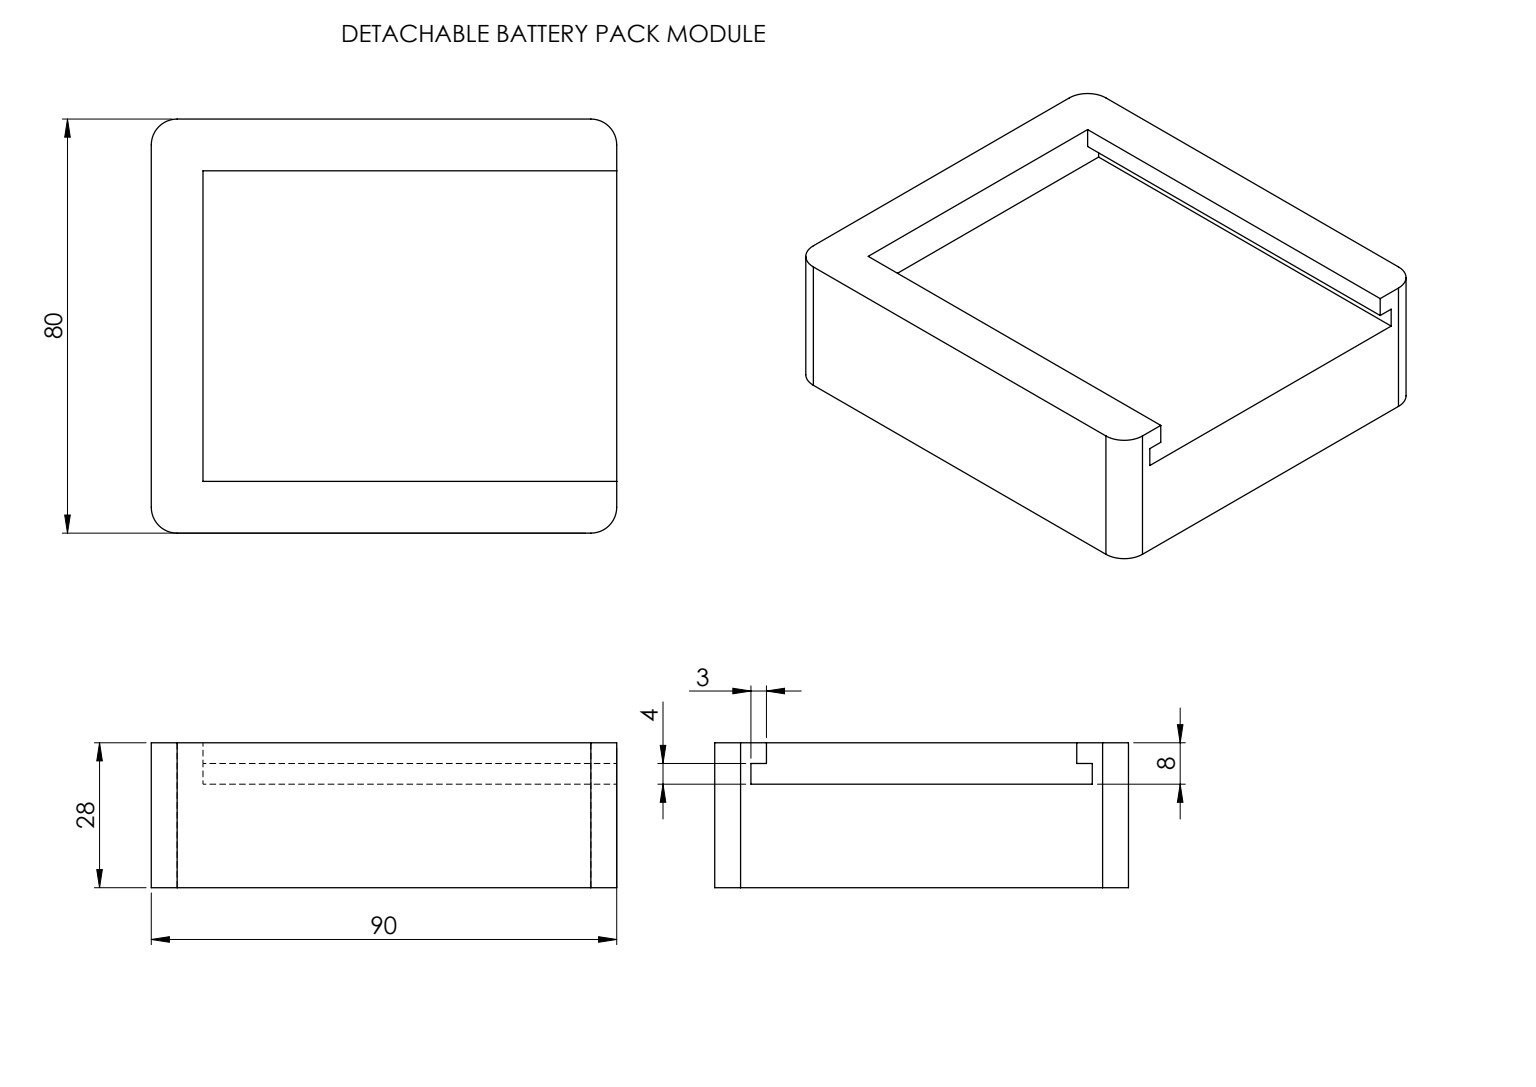
ISO-10303-21;
HEADER;
FILE_DESCRIPTION (('STEP AP214'),
    '1' );
FILE_NAME ('Detachable Battery Pack Module.step',
    '2026-10-05T20:22:16',
    ( '' ),
    ( '' ),
    'SwSTEP 2.0',
    'SolidWorks 2026',
    '' );
FILE_SCHEMA (( 'AUTOMOTIVE_DESIGN' ));
ENDSEC;

DATA;
#27=ORIENTED_EDGE ( 'NONE', *, *, #8063, .T. ) ;
#29=DIRECTION ( 'NONE',  ( 0.000000000000000000, 1.000000000000000000, 0.000000000000000000 ) ) ;
#99=ORIENTED_EDGE ( 'NONE', *, *, #10624, .F. ) ;
#105=LINE ( 'NONE', #5601, #6122 ) ;
#109=DIRECTION ( 'NONE',  ( -0.000000000000000000, -1.000000000000000000, -0.000000000000000000 ) ) ;
#122=AXIS2_PLACEMENT_3D ( 'NONE', #11876, #6482, #6572 ) ;
#131=CARTESIAN_POINT ( 'NONE',  ( 39.99999999999998579, 5.659323622547703371E-16, -33.00000000000000000 ) ) ;
#171=CARTESIAN_POINT ( 'NONE',  ( -40.00000000000000000, 8.000000000000000000, -40.00000000000000000 ) ) ;
#177=DIRECTION ( 'NONE',  ( 0.000000000000000000, -1.000000000000000000, 0.000000000000000000 ) ) ;
#268=CARTESIAN_POINT ( 'NONE',  ( 34.99999999999999289, -20.00000000000000000, 39.99999999999998579 ) ) ;
#302=EDGE_CURVE ( 'NONE', #14819, #8809, #14878, .T. ) ;
#471=LINE ( 'NONE', #14027, #16068 ) ;
#480=ORIENTED_EDGE ( 'NONE', *, *, #11200, .F. ) ;
#487=AXIS2_PLACEMENT_3D ( 'NONE', #11537, #16029, #3909 ) ;
#495=EDGE_LOOP ( 'NONE', ( #13630, #14725, #1232, #7431, #16585, #10286, #6595, #15301, #1355, #7450, #11318, #10338 ) ) ;
#526=CARTESIAN_POINT ( 'NONE',  ( 39.99999999999998579, 4.000000000000000000, -33.00000000000000000 ) ) ;
#535=EDGE_LOOP ( 'NONE', ( #5840, #7471, #16377, #3579 ) ) ;
#604=LINE ( 'NONE', #8649, #6198 ) ;
#612=EDGE_CURVE ( 'NONE', #8809, #13930, #10178, .T. ) ;
#644=ORIENTED_EDGE ( 'NONE', *, *, #1969, .F. ) ;
#648=DIRECTION ( 'NONE',  ( 8.673617379884037937E-17, -2.891205793294676354E-16, -1.000000000000000000 ) ) ;
#666=CARTESIAN_POINT ( 'NONE',  ( 39.99999999999998579, 4.000000000000000000, -33.00000000000000000 ) ) ;
#672=ORIENTED_EDGE ( 'NONE', *, *, #16461, .F. ) ;
#689=ADVANCED_FACE ( 'NONE', ( #14335 ), #14508, .T. ) ;
#753=CARTESIAN_POINT ( 'NONE',  ( -44.99999999999997868, -20.00000000000000000, 40.00000000000000711 ) ) ;
#760=AXIS2_PLACEMENT_3D ( 'NONE', #526, #3591, #2173 ) ;
#772=DIRECTION ( 'NONE',  ( -0.000000000000000000, -0.000000000000000000, 1.000000000000000000 ) ) ;
#803=( GEOMETRIC_REPRESENTATION_CONTEXT ( 3 ) GLOBAL_UNCERTAINTY_ASSIGNED_CONTEXT ( ( #9704 ) ) GLOBAL_UNIT_ASSIGNED_CONTEXT ( ( #12385, #1419, #6983 ) ) REPRESENTATION_CONTEXT ( 'NONE', 'WORKASPACE' ) );
#850=AXIS2_PLACEMENT_3D ( 'NONE', #4169, #5324, #16475 ) ;
#851=DIRECTION ( 'NONE',  ( 0.000000000000000000, -2.891205793294676354E-16, -1.000000000000000000 ) ) ;
#864=CARTESIAN_POINT ( 'NONE',  ( 39.99999999999998579, 4.000000000000000000, -33.00000000000000000 ) ) ;
#880=CARTESIAN_POINT ( 'NONE',  ( -45.00000000000000711, -20.00000000000000000, -40.00000000000000000 ) ) ;
#899=DIRECTION ( 'NONE',  ( -0.000000000000000000, -1.000000000000000000, -0.000000000000000000 ) ) ;
#925=VERTEX_POINT ( 'NONE', #11652 ) ;
#980=CARTESIAN_POINT ( 'NONE',  ( -45.00000000000001421, -20.00000000000000000, 35.00000000000000711 ) ) ;
#982=FACE_OUTER_BOUND ( 'NONE', #16917, .T. ) ;
#1076=DIRECTION ( 'NONE',  ( -1.000000000000000000, 0.000000000000000000, -8.673617379884037937E-17 ) ) ;
#1155=DIRECTION ( 'NONE',  ( 0.000000000000000000, 1.000000000000000000, 0.000000000000000000 ) ) ;
#1187=EDGE_LOOP ( 'NONE', ( #2373, #9713, #10320, #7062, #15674, #5505, #13725, #7217, #5355, #10451, #13582, #2814 ) ) ;
#1204=DIRECTION ( 'NONE',  ( -0.000000000000000000, -0.000000000000000000, 1.000000000000000000 ) ) ;
#1232=ORIENTED_EDGE ( 'NONE', *, *, #3927, .T. ) ;
#1260=AXIS2_PLACEMENT_3D ( 'NONE', #15232, #14882, #16485 ) ;
#1263=CARTESIAN_POINT ( 'NONE',  ( 34.99999999999999289, -20.00000000000000000, -35.00000000000002132 ) ) ;
#1338=CARTESIAN_POINT ( 'NONE',  ( -40.00000000000000000, 8.000000000000007105, 30.00000000000000355 ) ) ;
#1355=ORIENTED_EDGE ( 'NONE', *, *, #6344, .T. ) ;
#1372=STYLED_ITEM ( 'NONE', ( #12556 ), #2569 ) ;
#1419=( NAMED_UNIT ( * ) PLANE_ANGLE_UNIT ( ) SI_UNIT ( $, .RADIAN. ) );
#1423=DIRECTION ( 'NONE',  ( 0.000000000000000000, -0.000000000000000000, 1.000000000000000000 ) ) ;
#1424=EDGE_CURVE ( 'NONE', #8476, #8508, #15662, .T. ) ;
#1428=CYLINDRICAL_SURFACE ( 'NONE', #7596, 4.999999999999997335 ) ;
#1453=ORIENTED_EDGE ( 'NONE', *, *, #6083, .T. ) ;
#1481=VERTEX_POINT ( 'NONE', #4870 ) ;
#1498=DIRECTION ( 'NONE',  ( -1.000000000000000000, 0.000000000000000000, 0.000000000000000000 ) ) ;
#1510=EDGE_LOOP ( 'NONE', ( #13211, #4341, #7022, #15878, #8880, #5058, #3959, #10219 ) ) ;
#1555=LINE ( 'NONE', #12356, #6673 ) ;
#1556=ORIENTED_EDGE ( 'NONE', *, *, #1424, .F. ) ;
#1565=( NAMED_UNIT ( * ) SI_UNIT ( $, .STERADIAN. ) SOLID_ANGLE_UNIT ( ) );
#1585=CLOSED_SHELL ( 'NONE', ( #12508, #15158, #17233, #3535, #8065, #16357, #12591, #1655, #12803, #4422, #689, #10482, #7807, #15850, #9522, #5248, #16253, #9807 ) ) ;
#1655=ADVANCED_FACE ( 'NONE', ( #13541 ), #14946, .T. ) ;
#1662=VECTOR ( 'NONE', #12747, 1000.000000000000000 ) ;
#1663=SURFACE_STYLE_USAGE ( .BOTH. , #5645 ) ;
#1694=VECTOR ( 'NONE', #11931, 1000.000000000000000 ) ;
#1696=VERTEX_POINT ( 'NONE', #8098 ) ;
#1698=VECTOR ( 'NONE', #6202, 1000.000000000000000 ) ;
#1747=( NAMED_UNIT ( * ) PLANE_ANGLE_UNIT ( ) SI_UNIT ( $, .RADIAN. ) );
#1761=FILL_AREA_STYLE ('',( #3087 ) ) ;
#1803=VERTEX_POINT ( 'NONE', #3052 ) ;
#1804=PLANE ( 'NONE',  #16988 ) ;
#1855=EDGE_CURVE ( 'NONE', #11143, #17364, #4482, .T. ) ;
#1857=CARTESIAN_POINT ( 'NONE',  ( 39.99999999999998579, 4.000000000000007994, 33.00000000000001421 ) ) ;
#1893=DIRECTION ( 'NONE',  ( 6.938893903907229364E-16, -0.000000000000000000, -1.000000000000000000 ) ) ;
#1955=EDGE_CURVE ( 'NONE', #4989, #2572, #9262, .T. ) ;
#1969=EDGE_CURVE ( 'NONE', #1803, #9465, #6493, .T. ) ;
#2096=LINE ( 'NONE', #16729, #17441 ) ;
#2142=CARTESIAN_POINT ( 'NONE',  ( -40.00000000000000000, 4.000000000000007105, 30.00000000000000711 ) ) ;
#2173=DIRECTION ( 'NONE',  ( 1.000000000000000000, 0.000000000000000000, 8.673617379884037937E-17 ) ) ;
#2179=CARTESIAN_POINT ( 'NONE',  ( 34.99999999999999289, -20.00000000000000000, -40.00000000000001421 ) ) ;
#2196=LINE ( 'NONE', #880, #4743 ) ;
#2208=VERTEX_POINT ( 'NONE', #16049 ) ;
#2216=CARTESIAN_POINT ( 'NONE',  ( 39.99999999999997868, 8.000000000000010658, 40.00000000000000711 ) ) ;
#2243=AXIS2_PLACEMENT_3D ( 'NONE', #5868, #9754, #1076 ) ;
#2254=AXIS2_PLACEMENT_3D ( 'NONE', #12118, #6975, #8121 ) ;
#2256=VECTOR ( 'NONE', #10322, 1000.000000000000000 ) ;
#2373=ORIENTED_EDGE ( 'NONE', *, *, #6135, .T. ) ;
#2437=CARTESIAN_POINT ( 'NONE',  ( -44.99999999999998579, 8.000000000000010658, 40.00000000000000000 ) ) ;
#2452=EDGE_CURVE ( 'NONE', #9465, #8476, #4703, .T. ) ;
#2492=ORIENTED_EDGE ( 'NONE', *, *, #1855, .F. ) ;
#2498=EDGE_CURVE ( 'NONE', #10657, #14819, #17440, .T. ) ;
#2512=VECTOR ( 'NONE', #14109, 1000.000000000000000 ) ;
#2523=AXIS2_PLACEMENT_3D ( 'NONE', #6254, #15465, #11391 ) ;
#2541=DIRECTION ( 'NONE',  ( -1.000000000000000000, 0.000000000000000000, -8.673617379884037937E-17 ) ) ;
#2550=CARTESIAN_POINT ( 'NONE',  ( -40.00000000000000000, 4.000000000000000000, -33.00000000000000711 ) ) ;
#2569=ADVANCED_BREP_SHAPE_REPRESENTATION ( '', ( #5314, #3583 ), #803 ) ;
#2572=VERTEX_POINT ( 'NONE', #11945 ) ;
#2585=DIRECTION ( 'NONE',  ( 0.000000000000000000, 1.000000000000000000, 0.000000000000000000 ) ) ;
#2603=DIRECTION ( 'NONE',  ( -0.000000000000000000, -1.000000000000000000, -0.000000000000000000 ) ) ;
#2660=LINE ( 'NONE', #171, #7546 ) ;
#2662=DIRECTION ( 'NONE',  ( 7.523163845262643335E-32, 1.000000000000000000, -8.673617379884037444E-16 ) ) ;
#2671=CYLINDRICAL_SURFACE ( 'NONE', #122, 5.000000000000000888 ) ;
#2717=VERTEX_POINT ( 'NONE', #6180 ) ;
#2814=ORIENTED_EDGE ( 'NONE', *, *, #9455, .T. ) ;
#2848=EDGE_CURVE ( 'NONE', #1696, #5755, #4931, .T. ) ;
#2887=EDGE_LOOP ( 'NONE', ( #13403, #3178, #13306, #5990 ) ) ;
#2973=VERTEX_POINT ( 'NONE', #15019 ) ;
#2981=ORIENTED_EDGE ( 'NONE', *, *, #16182, .T. ) ;
#3052=CARTESIAN_POINT ( 'NONE',  ( 39.99999999999999289, 8.000000000000000000, -35.00000000000002132 ) ) ;
#3087=FILL_AREA_STYLE_COLOUR ( '', #9802 ) ;
#3137=CARTESIAN_POINT ( 'NONE',  ( 39.99999999999998579, 8.000000000000007105, 30.00000000000001066 ) ) ;
#3141=DIRECTION ( 'NONE',  ( 0.000000000000000000, 2.891205793294675861E-16, 1.000000000000000000 ) ) ;
#3178=ORIENTED_EDGE ( 'NONE', *, *, #4303, .T. ) ;
#3219=FACE_OUTER_BOUND ( 'NONE', #535, .T. ) ;
#3239=ORIENTED_EDGE ( 'NONE', *, *, #6135, .F. ) ;
#3258=DIRECTION ( 'NONE',  ( 0.000000000000000000, 1.000000000000000000, 0.000000000000000000 ) ) ;
#3274=AXIS2_PLACEMENT_3D ( 'NONE', #5480, #1498, #8297 ) ;
#3307=AXIS2_PLACEMENT_3D ( 'NONE', #15748, #14596, #11938 ) ;
#3435=AXIS2_PLACEMENT_3D ( 'NONE', #1263, #10821, #5163 ) ;
#3464=DIRECTION ( 'NONE',  ( 6.938893903907229364E-16, -3.469446951953614682E-16, -1.000000000000000000 ) ) ;
#3477=DIRECTION ( 'NONE',  ( 1.000000000000000000, -0.000000000000000000, -2.312964634635742957E-16 ) ) ;
#3504=PLANE ( 'NONE',  #14956 ) ;
#3535=ADVANCED_FACE ( 'NONE', ( #3219 ), #1804, .T. ) ;
#3546=STYLED_ITEM ( 'NONE', ( #13619 ), #5314 ) ;
#3557=EDGE_CURVE ( 'NONE', #13930, #11460, #471, .T. ) ;
#3564=EDGE_LOOP ( 'NONE', ( #3924, #13589, #644, #3850 ) ) ;
#3579=ORIENTED_EDGE ( 'NONE', *, *, #11915, .T. ) ;
#3583=AXIS2_PLACEMENT_3D ( 'NONE', #5482, #6893, #8222 ) ;
#3585=VECTOR ( 'NONE', #8683, 1000.000000000000000 ) ;
#3586=ORIENTED_EDGE ( 'NONE', *, *, #13440, .T. ) ;
#3591=DIRECTION ( 'NONE',  ( -8.673617379884037937E-17, 0.000000000000000000, 1.000000000000000000 ) ) ;
#3596=FACE_OUTER_BOUND ( 'NONE', #10262, .T. ) ;
#3619=LINE ( 'NONE', #5122, #7835 ) ;
#3640=LINE ( 'NONE', #2216, #3874 ) ;
#3684=PLANE ( 'NONE',  #760 ) ;
#3689=DIRECTION ( 'NONE',  ( -1.000000000000000000, 0.000000000000000000, -8.673617379884037937E-17 ) ) ;
#3703=FACE_OUTER_BOUND ( 'NONE', #6699, .T. ) ;
#3717=ORIENTED_EDGE ( 'NONE', *, *, #14584, .T. ) ;
#3777=CARTESIAN_POINT ( 'NONE',  ( 34.99999999999999289, 8.000000000000000000, -35.00000000000002132 ) ) ;
#3850=ORIENTED_EDGE ( 'NONE', *, *, #16742, .F. ) ;
#3851=DIRECTION ( 'NONE',  ( -2.507721281754210796E-32, -1.000000000000000000, 2.891205793294676354E-16 ) ) ;
#3874=VECTOR ( 'NONE', #3464, 1000.000000000000000 ) ;
#3897=PRODUCT_DEFINITION_FORMATION_WITH_SPECIFIED_SOURCE ( 'ANY', '', #15498, .NOT_KNOWN. ) ;
#3899=AXIS2_PLACEMENT_3D ( 'NONE', #14295, #3851, #851 ) ;
#3909=DIRECTION ( 'NONE',  ( -1.000000000000000000, 0.000000000000000000, 1.541976423090495387E-16 ) ) ;
#3913=( GEOMETRIC_REPRESENTATION_CONTEXT ( 3 ) GLOBAL_UNCERTAINTY_ASSIGNED_CONTEXT ( ( #4233 ) ) GLOBAL_UNIT_ASSIGNED_CONTEXT ( ( #5828, #12646, #4678 ) ) REPRESENTATION_CONTEXT ( 'NONE', 'WORKASPACE' ) );
#3924=ORIENTED_EDGE ( 'NONE', *, *, #7277, .F. ) ;
#3927=EDGE_CURVE ( 'NONE', #9465, #10480, #11324, .T. ) ;
#3959=ORIENTED_EDGE ( 'NONE', *, *, #7710, .F. ) ;
#3993=EDGE_CURVE ( 'NONE', #9130, #2572, #15479, .T. ) ;
#4021=ORIENTED_EDGE ( 'NONE', *, *, #11179, .T. ) ;
#4158=ORIENTED_EDGE ( 'NONE', *, *, #16909, .F. ) ;
#4169=CARTESIAN_POINT ( 'NONE',  ( 39.99999999999999289, 8.000000000000000000, -39.99999999999999289 ) ) ;
#4201=VERTEX_POINT ( 'NONE', #15021 ) ;
#4207=ORIENTED_EDGE ( 'NONE', *, *, #6451, .F. ) ;
#4233=UNCERTAINTY_MEASURE_WITH_UNIT (LENGTH_MEASURE( 1.000000000000000082E-05 ), #5828, 'distance_accuracy_value', 'NONE');
#4303=EDGE_CURVE ( 'NONE', #5755, #2973, #16626, .T. ) ;
#4321=DIRECTION ( 'NONE',  ( 0.000000000000000000, 0.000000000000000000, -1.000000000000000000 ) ) ;
#4341=ORIENTED_EDGE ( 'NONE', *, *, #11729, .F. ) ;
#4365=PLANE ( 'NONE',  #2243 ) ;
#4421=VERTEX_POINT ( 'NONE', #5908 ) ;
#4422=ADVANCED_FACE ( 'NONE', ( #10229 ), #3504, .T. ) ;
#4482=LINE ( 'NONE', #6952, #6475 ) ;
#4575=ORIENTED_EDGE ( 'NONE', *, *, #15298, .T. ) ;
#4647=CARTESIAN_POINT ( 'NONE',  ( -50.00000000000000711, -20.00000000000000000, 35.00000000000000711 ) ) ;
#4678=( NAMED_UNIT ( * ) SI_UNIT ( $, .STERADIAN. ) SOLID_ANGLE_UNIT ( ) );
#4703=LINE ( 'NONE', #10092, #1698 ) ;
#4743=VECTOR ( 'NONE', #5559, 1000.000000000000000 ) ;
#4870=CARTESIAN_POINT ( 'NONE',  ( 39.99999999999998579, -20.00000000000000000, -35.00000000000002132 ) ) ;
#4902=DIRECTION ( 'NONE',  ( 0.000000000000000000, -1.000000000000000000, 8.673617379884035472E-16 ) ) ;
#4913=FACE_OUTER_BOUND ( 'NONE', #12663, .T. ) ;
#4931=LINE ( 'NONE', #14765, #2256 ) ;
#4958=CARTESIAN_POINT ( 'NONE',  ( 34.99999999999999289, 8.000000000000000000, 34.99999999999999289 ) ) ;
#4970=ORIENTED_EDGE ( 'NONE', *, *, #11200, .T. ) ;
#4988=CARTESIAN_POINT ( 'NONE',  ( 39.99999999999998579, 8.000000000000000000, -29.99999999999999645 ) ) ;
#4989=VERTEX_POINT ( 'NONE', #10096 ) ;
#5058=ORIENTED_EDGE ( 'NONE', *, *, #12886, .F. ) ;
#5108=EDGE_CURVE ( 'NONE', #13611, #8508, #7764, .T. ) ;
#5122=CARTESIAN_POINT ( 'NONE',  ( 39.99999999999997868, 8.000000000000010658, 40.00000000000000711 ) ) ;
#5126=EDGE_CURVE ( 'NONE', #17364, #16020, #16555, .T. ) ;
#5145=DIRECTION ( 'NONE',  ( 0.000000000000000000, 0.000000000000000000, 1.000000000000000000 ) ) ;
#5152=ORIENTED_EDGE ( 'NONE', *, *, #13297, .T. ) ;
#5163=DIRECTION ( 'NONE',  ( 0.000000000000000000, 0.000000000000000000, 1.000000000000000000 ) ) ;
#5199=ORIENTED_EDGE ( 'NONE', *, *, #16103, .T. ) ;
#5248=ADVANCED_FACE ( 'NONE', ( #3703 ), #6537, .T. ) ;
#5313=DIRECTION ( 'NONE',  ( -0.000000000000000000, -1.000000000000000000, -0.000000000000000000 ) ) ;
#5314=MANIFOLD_SOLID_BREP ( 'Fillet1', #1585 ) ;
#5324=DIRECTION ( 'NONE',  ( 0.000000000000000000, 1.000000000000000000, 0.000000000000000000 ) ) ;
#5355=ORIENTED_EDGE ( 'NONE', *, *, #9268, .F. ) ;
#5434=ORIENTED_EDGE ( 'NONE', *, *, #8492, .F. ) ;
#5480=CARTESIAN_POINT ( 'NONE',  ( -50.00000000000000711, -20.00000000000000000, 40.00000000000000711 ) ) ;
#5482=CARTESIAN_POINT ( 'NONE',  ( 0.000000000000000000, 0.000000000000000000, 0.000000000000000000 ) ) ;
#5505=ORIENTED_EDGE ( 'NONE', *, *, #14789, .F. ) ;
#5559=DIRECTION ( 'NONE',  ( 0.000000000000000000, 1.000000000000000000, 0.000000000000000000 ) ) ;
#5582=ORIENTED_EDGE ( 'NONE', *, *, #10226, .T. ) ;
#5601=CARTESIAN_POINT ( 'NONE',  ( -40.00000000000000000, 4.000000000000007994, 33.00000000000000711 ) ) ;
#5621=PRODUCT_CONTEXT ( 'NONE', #8225, 'mechanical' ) ;
#5645=SURFACE_SIDE_STYLE ('',( #13694 ) ) ;
#5662=SURFACE_STYLE_FILL_AREA ( #1761 ) ;
#5682=FACE_OUTER_BOUND ( 'NONE', #10377, .T. ) ;
#5747=PLANE ( 'NONE',  #6125 ) ;
#5755=VERTEX_POINT ( 'NONE', #11364 ) ;
#5828=( LENGTH_UNIT ( ) NAMED_UNIT ( * ) SI_UNIT ( .MILLI., .METRE. ) );
#5840=ORIENTED_EDGE ( 'NONE', *, *, #16909, .T. ) ;
#5863=VECTOR ( 'NONE', #17323, 1000.000000000000000 ) ;
#5868=CARTESIAN_POINT ( 'NONE',  ( 39.99999999999998579, 4.000000000000007994, 33.00000000000001421 ) ) ;
#5871=CARTESIAN_POINT ( 'NONE',  ( 39.99999999999998579, 8.000000000000008882, 34.99999999999999289 ) ) ;
#5908=CARTESIAN_POINT ( 'NONE',  ( 39.99999999999998579, 4.000000000000000000, -30.00000000000000000 ) ) ;
#5990=ORIENTED_EDGE ( 'NONE', *, *, #12095, .T. ) ;
#6083=EDGE_CURVE ( 'NONE', #6776, #925, #105, .T. ) ;
#6122=VECTOR ( 'NONE', #29, 1000.000000000000000 ) ;
#6125=AXIS2_PLACEMENT_3D ( 'NONE', #12216, #13906, #1423 ) ;
#6135=EDGE_CURVE ( 'NONE', #2717, #1481, #9571, .T. ) ;
#6142=LINE ( 'NONE', #17472, #15017 ) ;
#6180=CARTESIAN_POINT ( 'NONE',  ( 39.99999999999998579, -20.00000000000000000, 34.99999999999999289 ) ) ;
#6198=VECTOR ( 'NONE', #772, 1000.000000000000000 ) ;
#6202=DIRECTION ( 'NONE',  ( -0.000000000000000000, -1.000000000000000000, -0.000000000000000000 ) ) ;
#6254=CARTESIAN_POINT ( 'NONE',  ( 0.000000000000000000, -20.00000000000000000, 0.000000000000000000 ) ) ;
#6280=CARTESIAN_POINT ( 'NONE',  ( 39.99999999999998579, 8.648601236627303230E-15, 33.00000000000001421 ) ) ;
#6344=EDGE_CURVE ( 'NONE', #16020, #15739, #3640, .T. ) ;
#6420=DIRECTION ( 'NONE',  ( -1.000000000000000000, 0.000000000000000000, -8.673617379884036705E-17 ) ) ;
#6425=LINE ( 'NONE', #864, #14159 ) ;
#6451=EDGE_CURVE ( 'NONE', #13930, #10657, #13763, .T. ) ;
#6465=VECTOR ( 'NONE', #7501, 1000.000000000000000 ) ;
#6475=VECTOR ( 'NONE', #9778, 1000.000000000000000 ) ;
#6482=DIRECTION ( 'NONE',  ( 0.000000000000000000, 1.000000000000000000, 0.000000000000000000 ) ) ;
#6493=CIRCLE ( 'NONE', #16405, 5.000000000000000888 ) ;
#6504=FACE_OUTER_BOUND ( 'NONE', #13919, .T. ) ;
#6513=PLANE ( 'NONE',  #16560 ) ;
#6537=CYLINDRICAL_SURFACE ( 'NONE', #7777, 4.999999999999997335 ) ;
#6572=DIRECTION ( 'NONE',  ( 0.000000000000000000, 0.000000000000000000, 1.000000000000000000 ) ) ;
#6595=ORIENTED_EDGE ( 'NONE', *, *, #13297, .F. ) ;
#6628=LINE ( 'NONE', #11930, #10435 ) ;
#6673=VECTOR ( 'NONE', #16260, 1000.000000000000000 ) ;
#6685=ORIENTED_EDGE ( 'NONE', *, *, #1424, .T. ) ;
#6699=EDGE_LOOP ( 'NONE', ( #11829, #13069, #8413, #2492 ) ) ;
#6717=ORIENTED_EDGE ( 'NONE', *, *, #16182, .F. ) ;
#6763=FACE_OUTER_BOUND ( 'NONE', #3564, .T. ) ;
#6776=VERTEX_POINT ( 'NONE', #14079 ) ;
#6893=DIRECTION ( 'NONE',  ( 0.000000000000000000, 0.000000000000000000, 1.000000000000000000 ) ) ;
#6904=VECTOR ( 'NONE', #3477, 1000.000000000000000 ) ;
#6906=DIRECTION ( 'NONE',  ( 0.000000000000000000, 1.000000000000000000, 0.000000000000000000 ) ) ;
#6928=AXIS2_PLACEMENT_3D ( 'NONE', #8934, #899, #10188 ) ;
#6947=VECTOR ( 'NONE', #648, 1000.000000000000000 ) ;
#6952=CARTESIAN_POINT ( 'NONE',  ( 34.99999999999999289, -20.00000000000000000, 39.99999999999998579 ) ) ;
#6956=PRODUCT_DEFINITION_CONTEXT ( 'detailed design', #9124, 'design' ) ;
#6975=DIRECTION ( 'NONE',  ( -8.673617379884036705E-17, -8.673617379884037444E-16, 1.000000000000000000 ) ) ;
#6983=( NAMED_UNIT ( * ) SI_UNIT ( $, .STERADIAN. ) SOLID_ANGLE_UNIT ( ) );
#7022=ORIENTED_EDGE ( 'NONE', *, *, #1955, .F. ) ;
#7040=CARTESIAN_POINT ( 'NONE',  ( 39.99999999999998579, 4.000000000000007105, 30.00000000000001421 ) ) ;
#7048=CARTESIAN_POINT ( 'NONE',  ( -40.00000000000000000, 4.000000000000007105, 30.00000000000000711 ) ) ;
#7062=ORIENTED_EDGE ( 'NONE', *, *, #12095, .F. ) ;
#7122=DIRECTION ( 'NONE',  ( 0.000000000000000000, 1.000000000000000000, -8.673617379884037444E-16 ) ) ;
#7158=SURFACE_STYLE_USAGE ( .BOTH. , #16468 ) ;
#7189=FACE_OUTER_BOUND ( 'NONE', #16403, .T. ) ;
#7217=ORIENTED_EDGE ( 'NONE', *, *, #11179, .F. ) ;
#7241=VERTEX_POINT ( 'NONE', #10994 ) ;
#7277=EDGE_CURVE ( 'NONE', #8476, #1481, #9445, .T. ) ;
#7322=ORIENTED_EDGE ( 'NONE', *, *, #2498, .T. ) ;
#7336=SHAPE_REPRESENTATION_RELATIONSHIP ( 'NONE' , 'NONE' ,  #17073, #2569 ) ;
#7348=LINE ( 'NONE', #1857, #11171 ) ;
#7431=ORIENTED_EDGE ( 'NONE', *, *, #15495, .T. ) ;
#7450=ORIENTED_EDGE ( 'NONE', *, *, #14565, .T. ) ;
#7451=LINE ( 'NONE', #12688, #6904 ) ;
#7467=CARTESIAN_POINT ( 'NONE',  ( 39.99999999999998579, 4.000000000000007105, 30.00000000000001421 ) ) ;
#7471=ORIENTED_EDGE ( 'NONE', *, *, #7710, .T. ) ;
#7501=DIRECTION ( 'NONE',  ( -1.000000000000000000, 0.000000000000000000, -8.673617379884037937E-17 ) ) ;
#7521=VECTOR ( 'NONE', #4902, 1000.000000000000000 ) ;
#7527=DIRECTION ( 'NONE',  ( 0.000000000000000000, 0.000000000000000000, 1.000000000000000000 ) ) ;
#7532=VECTOR ( 'NONE', #8248, 1000.000000000000000 ) ;
#7546=VECTOR ( 'NONE', #16213, 1000.000000000000000 ) ;
#7596=AXIS2_PLACEMENT_3D ( 'NONE', #13196, #2585, #5145 ) ;
#7600=CARTESIAN_POINT ( 'NONE',  ( 39.99999999999998579, 4.000000000000007994, 33.00000000000001421 ) ) ;
#7607=CARTESIAN_POINT ( 'NONE',  ( 39.99999999999998579, -20.00000000000000000, -40.00000000000001421 ) ) ;
#7710=EDGE_CURVE ( 'NONE', #14757, #7241, #12139, .T. ) ;
#7720=CARTESIAN_POINT ( 'NONE',  ( -50.00000000000005684, 8.000000000000000000, 35.00000000000000711 ) ) ;
#7747=LINE ( 'NONE', #12003, #13159 ) ;
#7764=CIRCLE ( 'NONE', #6928, 5.000000000000000888 ) ;
#7767=CIRCLE ( 'NONE', #10318, 5.000000000000000888 ) ;
#7775=CARTESIAN_POINT ( 'NONE',  ( -45.00000000000000711, -20.00000000000000000, 40.00000000000000711 ) ) ;
#7777=AXIS2_PLACEMENT_3D ( 'NONE', #9270, #15998, #9090 ) ;
#7807=ADVANCED_FACE ( 'NONE', ( #10881 ), #14872, .T. ) ;
#7835=VECTOR ( 'NONE', #13089, 1000.000000000000000 ) ;
#7858=CARTESIAN_POINT ( 'NONE',  ( -40.00000000000000000, 4.000000000000000000, -30.00000000000000711 ) ) ;
#7989=CYLINDRICAL_SURFACE ( 'NONE', #3435, 5.000000000000000888 ) ;
#8063=EDGE_CURVE ( 'NONE', #2973, #4989, #17250, .T. ) ;
#8065=ADVANCED_FACE ( 'NONE', ( #13270 ), #10252, .T. ) ;
#8098=CARTESIAN_POINT ( 'NONE',  ( 39.99999999999998579, 8.000000000000000000, -29.99999999999999645 ) ) ;
#8121=DIRECTION ( 'NONE',  ( 0.000000000000000000, -1.000000000000000000, -8.673617379884037444E-16 ) ) ;
#8153=ORIENTED_EDGE ( 'NONE', *, *, #2452, .T. ) ;
#8222=DIRECTION ( 'NONE',  ( 1.000000000000000000, 0.000000000000000000, 0.000000000000000000 ) ) ;
#8225=APPLICATION_CONTEXT ( 'automotive_design' ) ;
#8248=DIRECTION ( 'NONE',  ( 0.000000000000000000, 0.000000000000000000, -1.000000000000000000 ) ) ;
#8288=FILL_AREA_STYLE ('',( #13887 ) ) ;
#8297=DIRECTION ( 'NONE',  ( 0.000000000000000000, 0.000000000000000000, 1.000000000000000000 ) ) ;
#8413=ORIENTED_EDGE ( 'NONE', *, *, #5126, .F. ) ;
#8461=ORIENTED_EDGE ( 'NONE', *, *, #7277, .T. ) ;
#8472=( LENGTH_UNIT ( ) NAMED_UNIT ( * ) SI_UNIT ( .MILLI., .METRE. ) );
#8476=VERTEX_POINT ( 'NONE', #2179 ) ;
#8492=EDGE_CURVE ( 'NONE', #2208, #4989, #6425, .T. ) ;
#8508=VERTEX_POINT ( 'NONE', #11649 ) ;
#8638=MECHANICAL_DESIGN_GEOMETRIC_PRESENTATION_REPRESENTATION('',(#3546),#10614);
#8645=DIRECTION ( 'NONE',  ( 0.000000000000000000, 0.000000000000000000, -1.000000000000000000 ) ) ;
#8649=CARTESIAN_POINT ( 'NONE',  ( -50.00000000000000711, -20.00000000000000000, 40.00000000000000711 ) ) ;
#8683=DIRECTION ( 'NONE',  ( -1.000000000000000000, 0.000000000000000000, -8.673617379884037937E-17 ) ) ;
#8809=VERTEX_POINT ( 'NONE', #4647 ) ;
#8851=DIRECTION ( 'NONE',  ( 0.000000000000000000, 1.000000000000000000, 0.000000000000000000 ) ) ;
#8866=ORIENTED_EDGE ( 'NONE', *, *, #9268, .T. ) ;
#8878=LINE ( 'NONE', #17035, #7521 ) ;
#8880=ORIENTED_EDGE ( 'NONE', *, *, #4303, .F. ) ;
#8934=CARTESIAN_POINT ( 'NONE',  ( -45.00000000000000711, -20.00000000000000000, -35.00000000000000000 ) ) ;
#8952=ORIENTED_EDGE ( 'NONE', *, *, #13345, .T. ) ;
#8978=ORIENTED_EDGE ( 'NONE', *, *, #612, .T. ) ;
#8999=VECTOR ( 'NONE', #16456, 1000.000000000000000 ) ;
#9015=ORIENTED_EDGE ( 'NONE', *, *, #5108, .F. ) ;
#9022=VECTOR ( 'NONE', #14341, 1000.000000000000000 ) ;
#9070=VECTOR ( 'NONE', #3141, 1000.000000000000000 ) ;
#9090=DIRECTION ( 'NONE',  ( 0.000000000000000000, 0.000000000000000000, 1.000000000000000000 ) ) ;
#9122=DIRECTION ( 'NONE',  ( -0.000000000000000000, -1.000000000000000000, -0.000000000000000000 ) ) ;
#9124=APPLICATION_CONTEXT ( 'automotive_design' ) ;
#9130=VERTEX_POINT ( 'NONE', #131 ) ;
#9155=FACE_OUTER_BOUND ( 'NONE', #1510, .T. ) ;
#9261=ORIENTED_EDGE ( 'NONE', *, *, #13345, .F. ) ;
#9262=LINE ( 'NONE', #2550, #16964 ) ;
#9268=EDGE_CURVE ( 'NONE', #11936, #15042, #13867, .T. ) ;
#9270=CARTESIAN_POINT ( 'NONE',  ( 34.99999999999999289, -20.00000000000000000, 34.99999999999999289 ) ) ;
#9324=DIRECTION ( 'NONE',  ( -0.000000000000000000, 1.000000000000000000, 8.673617379884035472E-16 ) ) ;
#9386=FACE_OUTER_BOUND ( 'NONE', #11761, .T. ) ;
#9445=CIRCLE ( 'NONE', #17381, 5.000000000000000888 ) ;
#9455=EDGE_CURVE ( 'NONE', #16020, #2717, #6142, .T. ) ;
#9465=VERTEX_POINT ( 'NONE', #16152 ) ;
#9478=ORIENTED_EDGE ( 'NONE', *, *, #3927, .F. ) ;
#9521=EDGE_LOOP ( 'NONE', ( #2981, #10816, #5152, #7322 ) ) ;
#9522=ADVANCED_FACE ( 'NONE', ( #6763 ), #7989, .T. ) ;
#9571=LINE ( 'NONE', #14976, #7532 ) ;
#9704=UNCERTAINTY_MEASURE_WITH_UNIT (LENGTH_MEASURE( 1.000000000000000082E-05 ), #12385, 'distance_accuracy_value', 'NONE');
#9713=ORIENTED_EDGE ( 'NONE', *, *, #16742, .T. ) ;
#9754=DIRECTION ( 'NONE',  ( 8.673617379884037937E-17, 0.000000000000000000, -1.000000000000000000 ) ) ;
#9778=DIRECTION ( 'NONE',  ( 0.000000000000000000, 1.000000000000000000, 0.000000000000000000 ) ) ;
#9779=DIRECTION ( 'NONE',  ( -0.000000000000000000, 1.000000000000000000, -0.000000000000000000 ) ) ;
#9802=COLOUR_RGB ( '', 0.09019608, 0.27058824, 0.51372549) ;
#9807=ADVANCED_FACE ( 'NONE', ( #9386 ), #1428, .T. ) ;
#9861=VECTOR ( 'NONE', #9779, 1000.000000000000000 ) ;
#9931=EDGE_LOOP ( 'NONE', ( #10239, #5582, #13958, #8978 ) ) ;
#10052=CARTESIAN_POINT ( 'NONE',  ( -44.99999999999997158, 8.000000000000000000, -40.00000000000000000 ) ) ;
#10055=CARTESIAN_POINT ( 'NONE',  ( -50.00000000000000000, 8.000000000000000000, -35.00000000000000000 ) ) ;
#10092=CARTESIAN_POINT ( 'NONE',  ( 34.99999999999999289, -20.00000000000000000, -40.00000000000001421 ) ) ;
#10096=CARTESIAN_POINT ( 'NONE',  ( -40.00000000000000000, 4.000000000000000000, -33.00000000000000711 ) ) ;
#10105=ORIENTED_EDGE ( 'NONE', *, *, #5108, .T. ) ;
#10111=CARTESIAN_POINT ( 'NONE',  ( 34.99999999999999289, 8.000000000000010658, 40.00000000000000711 ) ) ;
#10178=LINE ( 'NONE', #11338, #15163 ) ;
#10187=DIRECTION ( 'NONE',  ( 0.000000000000000000, 0.000000000000000000, 1.000000000000000000 ) ) ;
#10188=DIRECTION ( 'NONE',  ( 0.000000000000000000, 0.000000000000000000, 1.000000000000000000 ) ) ;
#10219=ORIENTED_EDGE ( 'NONE', *, *, #16103, .F. ) ;
#10226=EDGE_CURVE ( 'NONE', #11460, #13611, #6628, .T. ) ;
#10229=FACE_OUTER_BOUND ( 'NONE', #1187, .T. ) ;
#10239=ORIENTED_EDGE ( 'NONE', *, *, #3557, .T. ) ;
#10252=PLANE ( 'NONE',  #2254 ) ;
#10262=EDGE_LOOP ( 'NONE', ( #1556, #8461, #3239, #4575, #6717, #16679, #99, #10105 ) ) ;
#10286=ORIENTED_EDGE ( 'NONE', *, *, #6451, .T. ) ;
#10305=DIRECTION ( 'NONE',  ( -8.673617379884036705E-17, 0.000000000000000000, 1.000000000000000000 ) ) ;
#10308=CARTESIAN_POINT ( 'NONE',  ( -50.00000000000000711, -20.00000000000000000, -35.00000000000000000 ) ) ;
#10311=LINE ( 'NONE', #17052, #14657 ) ;
#10318=AXIS2_PLACEMENT_3D ( 'NONE', #10811, #6906, #11960 ) ;
#10320=ORIENTED_EDGE ( 'NONE', *, *, #11695, .F. ) ;
#10322=DIRECTION ( 'NONE',  ( -1.000000000000000000, 0.000000000000000000, -8.673617379884037937E-17 ) ) ;
#10338=ORIENTED_EDGE ( 'NONE', *, *, #2848, .F. ) ;
#10377=EDGE_LOOP ( 'NONE', ( #11379, #27, #5434, #3717 ) ) ;
#10435=VECTOR ( 'NONE', #14590, 1000.000000000000000 ) ;
#10451=ORIENTED_EDGE ( 'NONE', *, *, #11915, .F. ) ;
#10480=VERTEX_POINT ( 'NONE', #10052 ) ;
#10482=ADVANCED_FACE ( 'NONE', ( #3596 ), #14151, .F. ) ;
#10555=LINE ( 'NONE', #4988, #12904 ) ;
#10614=( GEOMETRIC_REPRESENTATION_CONTEXT ( 3 ) GLOBAL_UNCERTAINTY_ASSIGNED_CONTEXT ( ( #15888 ) ) GLOBAL_UNIT_ASSIGNED_CONTEXT ( ( #8472, #1747, #1565 ) ) REPRESENTATION_CONTEXT ( 'NONE', 'WORKASPACE' ) );
#10624=EDGE_CURVE ( 'NONE', #13611, #8809, #604, .T. ) ;
#10657=VERTEX_POINT ( 'NONE', #2437 ) ;
#10811=CARTESIAN_POINT ( 'NONE',  ( -45.00000000000000711, 8.000000000000000000, -35.00000000000000000 ) ) ;
#10816=ORIENTED_EDGE ( 'NONE', *, *, #1855, .T. ) ;
#10821=DIRECTION ( 'NONE',  ( 0.000000000000000000, 1.000000000000000000, 0.000000000000000000 ) ) ;
#10822=DIRECTION ( 'NONE',  ( 0.000000000000000000, 0.000000000000000000, 1.000000000000000000 ) ) ;
#10881=FACE_OUTER_BOUND ( 'NONE', #495, .T. ) ;
#10974=LINE ( 'NONE', #7600, #14564 ) ;
#10994=CARTESIAN_POINT ( 'NONE',  ( -40.00000000000000711, 8.000000000000000000, 30.00000000000000711 ) ) ;
#11052=ORIENTED_EDGE ( 'NONE', *, *, #1955, .T. ) ;
#11069=PLANE ( 'NONE',  #1260 ) ;
#11143=VERTEX_POINT ( 'NONE', #268 ) ;
#11171=VECTOR ( 'NONE', #177, 1000.000000000000000 ) ;
#11179=EDGE_CURVE ( 'NONE', #15042, #4201, #7348, .T. ) ;
#11200=EDGE_CURVE ( 'NONE', #15042, #925, #10974, .T. ) ;
#11318=ORIENTED_EDGE ( 'NONE', *, *, #12886, .T. ) ;
#11324=LINE ( 'NONE', #15569, #1662 ) ;
#11338=CARTESIAN_POINT ( 'NONE',  ( -50.00000000000000711, -20.00000000000000000, 35.00000000000000711 ) ) ;
#11354=CARTESIAN_POINT ( 'NONE',  ( 39.99999999999998579, 4.000000000000007994, 33.00000000000001421 ) ) ;
#11364=CARTESIAN_POINT ( 'NONE',  ( -40.00000000000000000, 8.000000000000000000, -30.00000000000000711 ) ) ;
#11379=ORIENTED_EDGE ( 'NONE', *, *, #15094, .T. ) ;
#11391=DIRECTION ( 'NONE',  ( 0.000000000000000000, -0.000000000000000000, 1.000000000000000000 ) ) ;
#11414=LINE ( 'NONE', #6280, #3585 ) ;
#11460=VERTEX_POINT ( 'NONE', #10055 ) ;
#11537=CARTESIAN_POINT ( 'NONE',  ( 39.99999999999998579, -20.00000000000000000, -40.00000000000001421 ) ) ;
#11649=CARTESIAN_POINT ( 'NONE',  ( -44.99999999999997868, -20.00000000000000000, -40.00000000000000000 ) ) ;
#11650=CARTESIAN_POINT ( 'NONE',  ( 39.99999999999998579, 8.000000000000007105, 30.00000000000001066 ) ) ;
#11652=CARTESIAN_POINT ( 'NONE',  ( -40.00000000000000000, 4.000000000000007994, 33.00000000000001421 ) ) ;
#11695=EDGE_CURVE ( 'NONE', #1696, #1803, #7747, .T. ) ;
#11729=EDGE_CURVE ( 'NONE', #2572, #6776, #1555, .T. ) ;
#11761=EDGE_LOOP ( 'NONE', ( #13734, #12081, #4207, #15357 ) ) ;
#11766=CARTESIAN_POINT ( 'NONE',  ( -45.00000000000001421, 8.000000000000000000, 35.00000000000000711 ) ) ;
#11829=ORIENTED_EDGE ( 'NONE', *, *, #15298, .F. ) ;
#11876=CARTESIAN_POINT ( 'NONE',  ( -45.00000000000000711, -20.00000000000000000, -35.00000000000000000 ) ) ;
#11915=EDGE_CURVE ( 'NONE', #15739, #11936, #8878, .T. ) ;
#11919=DIRECTION ( 'NONE',  ( 0.000000000000000000, 0.000000000000000000, 1.000000000000000000 ) ) ;
#11930=CARTESIAN_POINT ( 'NONE',  ( -50.00000000000000711, -20.00000000000000000, -35.00000000000000000 ) ) ;
#11931=DIRECTION ( 'NONE',  ( 8.673617379884037937E-17, 0.000000000000000000, -1.000000000000000000 ) ) ;
#11936=VERTEX_POINT ( 'NONE', #7467 ) ;
#11938=DIRECTION ( 'NONE',  ( 1.000000000000000000, 0.000000000000000000, -2.312964634635742957E-16 ) ) ;
#11945=CARTESIAN_POINT ( 'NONE',  ( -39.99999999999997158, 5.659323622547703371E-16, -33.00000000000000711 ) ) ;
#11960=DIRECTION ( 'NONE',  ( 0.000000000000000000, 0.000000000000000000, 1.000000000000000000 ) ) ;
#12003=CARTESIAN_POINT ( 'NONE',  ( 39.99999999999999289, 8.000000000000000000, -39.99999999999999289 ) ) ;
#12008=LINE ( 'NONE', #13257, #5863 ) ;
#12009=DIRECTION ( 'NONE',  ( 0.000000000000000000, -1.000000000000000000, 0.000000000000000000 ) ) ;
#12061=AXIS2_PLACEMENT_3D ( 'NONE', #11766, #8851, #10187 ) ;
#12081=ORIENTED_EDGE ( 'NONE', *, *, #2498, .F. ) ;
#12095=EDGE_CURVE ( 'NONE', #4421, #1696, #10555, .T. ) ;
#12118=CARTESIAN_POINT ( 'NONE',  ( 39.99999999999998579, 8.000000000000000000, -29.99999999999999645 ) ) ;
#12139=LINE ( 'NONE', #1338, #12158 ) ;
#12158=VECTOR ( 'NONE', #2662, 1000.000000000000000 ) ;
#12216=CARTESIAN_POINT ( 'NONE',  ( 0.000000000000000000, 0.000000000000000000, 0.000000000000000000 ) ) ;
#12239=CARTESIAN_POINT ( 'NONE',  ( 34.99999999999999289, -20.00000000000000000, -35.00000000000002132 ) ) ;
#12295=AXIS2_PLACEMENT_3D ( 'NONE', #4958, #1155, #7527 ) ;
#12356=CARTESIAN_POINT ( 'NONE',  ( -40.00000000000000000, 0.000000000000000000, -40.00000000000000000 ) ) ;
#12357=EDGE_LOOP ( 'NONE', ( #13174, #15785, #672, #3586 ) ) ;
#12385=( LENGTH_UNIT ( ) NAMED_UNIT ( * ) SI_UNIT ( .MILLI., .METRE. ) );
#12508=ADVANCED_FACE ( 'NONE', ( #16388 ), #5747, .T. ) ;
#12556=PRESENTATION_STYLE_ASSIGNMENT (( #7158 ) ) ;
#12591=ADVANCED_FACE ( 'NONE', ( #4913 ), #3684, .T. ) ;
#12614=LINE ( 'NONE', #666, #9861 ) ;
#12646=( NAMED_UNIT ( * ) PLANE_ANGLE_UNIT ( ) SI_UNIT ( $, .RADIAN. ) );
#12663=EDGE_LOOP ( 'NONE', ( #14472, #11052, #13504, #17338 ) ) ;
#12688=CARTESIAN_POINT ( 'NONE',  ( 39.99999999999998579, -20.00000000000000000, 39.99999999999998579 ) ) ;
#12747=DIRECTION ( 'NONE',  ( -1.000000000000000000, 0.000000000000000000, -8.673617379884037937E-17 ) ) ;
#12803=ADVANCED_FACE ( 'NONE', ( #12867 ), #14279, .T. ) ;
#12867=FACE_OUTER_BOUND ( 'NONE', #16398, .T. ) ;
#12886=EDGE_CURVE ( 'NONE', #7241, #5755, #2660, .T. ) ;
#12904=VECTOR ( 'NONE', #9324, 1000.000000000000000 ) ;
#12921=ORIENTED_EDGE ( 'NONE', *, *, #15495, .F. ) ;
#12980=CARTESIAN_POINT ( 'NONE',  ( 39.99999999999998579, -20.00000000000000000, 39.99999999999998579 ) ) ;
#13010=DIRECTION ( 'NONE',  ( -1.000000000000000000, 0.000000000000000000, -8.673617379884037937E-17 ) ) ;
#13069=ORIENTED_EDGE ( 'NONE', *, *, #9455, .F. ) ;
#13089=DIRECTION ( 'NONE',  ( -1.000000000000000000, 0.000000000000000000, -8.673617379884037937E-17 ) ) ;
#13147=CARTESIAN_POINT ( 'NONE',  ( -40.00000000000000711, 0.000000000000000000, -3.469446951953615767E-15 ) ) ;
#13159=VECTOR ( 'NONE', #17407, 1000.000000000000000 ) ;
#13174=ORIENTED_EDGE ( 'NONE', *, *, #3993, .T. ) ;
#13196=CARTESIAN_POINT ( 'NONE',  ( -45.00000000000001421, -20.00000000000000000, 35.00000000000000711 ) ) ;
#13211=ORIENTED_EDGE ( 'NONE', *, *, #6083, .F. ) ;
#13257=CARTESIAN_POINT ( 'NONE',  ( 39.99999999999998579, 4.000000000000007105, 30.00000000000001421 ) ) ;
#13270=FACE_OUTER_BOUND ( 'NONE', #2887, .T. ) ;
#13297=EDGE_CURVE ( 'NONE', #17364, #10657, #3619, .T. ) ;
#13306=ORIENTED_EDGE ( 'NONE', *, *, #15094, .F. ) ;
#13345=EDGE_CURVE ( 'NONE', #8508, #10480, #2196, .T. ) ;
#13403=ORIENTED_EDGE ( 'NONE', *, *, #2848, .T. ) ;
#13440=EDGE_CURVE ( 'NONE', #4201, #9130, #16458, .T. ) ;
#13504=ORIENTED_EDGE ( 'NONE', *, *, #3993, .F. ) ;
#13541=FACE_OUTER_BOUND ( 'NONE', #9931, .T. ) ;
#13582=ORIENTED_EDGE ( 'NONE', *, *, #6344, .F. ) ;
#13589=ORIENTED_EDGE ( 'NONE', *, *, #2452, .F. ) ;
#13595=SHAPE_DEFINITION_REPRESENTATION ( #16346, #17073 ) ;
#13611=VERTEX_POINT ( 'NONE', #10308 ) ;
#13619=PRESENTATION_STYLE_ASSIGNMENT (( #1663 ) ) ;
#13630=ORIENTED_EDGE ( 'NONE', *, *, #11695, .T. ) ;
#13694=SURFACE_STYLE_FILL_AREA ( #8288 ) ;
#13725=ORIENTED_EDGE ( 'NONE', *, *, #13440, .F. ) ;
#13734=ORIENTED_EDGE ( 'NONE', *, *, #302, .F. ) ;
#13753=LINE ( 'NONE', #16765, #2512 ) ;
#13763=CIRCLE ( 'NONE', #12061, 4.999999999999997335 ) ;
#13867=LINE ( 'NONE', #7040, #9070 ) ;
#13887=FILL_AREA_STYLE_COLOUR ( '', #17110 ) ;
#13906=DIRECTION ( 'NONE',  ( 0.000000000000000000, 1.000000000000000000, 0.000000000000000000 ) ) ;
#13919=EDGE_LOOP ( 'NONE', ( #4970, #5199, #4158, #8866 ) ) ;
#13930=VERTEX_POINT ( 'NONE', #7720 ) ;
#13958=ORIENTED_EDGE ( 'NONE', *, *, #10624, .T. ) ;
#13996=DIRECTION ( 'NONE',  ( 0.000000000000000000, 1.000000000000000000, 0.000000000000000000 ) ) ;
#14027=CARTESIAN_POINT ( 'NONE',  ( -50.00000000000000000, 8.000000000000000000, -40.00000000000000000 ) ) ;
#14079=CARTESIAN_POINT ( 'NONE',  ( -40.00000000000000711, 0.000000000000000000, 33.00000000000000711 ) ) ;
#14109=DIRECTION ( 'NONE',  ( -1.000000000000000000, 0.000000000000000000, -8.673617379884037937E-17 ) ) ;
#14151=PLANE ( 'NONE',  #2523 ) ;
#14159=VECTOR ( 'NONE', #3689, 1000.000000000000000 ) ;
#14194=CARTESIAN_POINT ( 'NONE',  ( 34.99999999999999289, -20.00000000000000000, 34.99999999999999289 ) ) ;
#14279=PLANE ( 'NONE',  #487 ) ;
#14295=CARTESIAN_POINT ( 'NONE',  ( 39.99999999999998579, 4.000000000000007105, 30.00000000000001421 ) ) ;
#14320=AXIS2_PLACEMENT_3D ( 'NONE', #980, #16140, #14718 ) ;
#14335=FACE_OUTER_BOUND ( 'NONE', #9521, .T. ) ;
#14341=DIRECTION ( 'NONE',  ( -1.000000000000000000, 0.000000000000000000, 1.541976423090495387E-16 ) ) ;
#14406=CIRCLE ( 'NONE', #16111, 4.999999999999997335 ) ;
#14472=ORIENTED_EDGE ( 'NONE', *, *, #8492, .T. ) ;
#14508=PLANE ( 'NONE',  #3307 ) ;
#14525=DIRECTION ( 'NONE',  ( 0.000000000000000000, 0.000000000000000000, 1.000000000000000000 ) ) ;
#14564=VECTOR ( 'NONE', #13010, 1000.000000000000000 ) ;
#14565=EDGE_CURVE ( 'NONE', #15739, #7241, #17134, .T. ) ;
#14584=EDGE_CURVE ( 'NONE', #2208, #4421, #10311, .T. ) ;
#14590=DIRECTION ( 'NONE',  ( -0.000000000000000000, -1.000000000000000000, -0.000000000000000000 ) ) ;
#14596=DIRECTION ( 'NONE',  ( 2.312964634635742957E-16, -0.000000000000000000, 1.000000000000000000 ) ) ;
#14657=VECTOR ( 'NONE', #1204, 1000.000000000000000 ) ;
#14718=DIRECTION ( 'NONE',  ( 0.000000000000000000, 0.000000000000000000, 1.000000000000000000 ) ) ;
#14725=ORIENTED_EDGE ( 'NONE', *, *, #1969, .T. ) ;
#14757=VERTEX_POINT ( 'NONE', #7048 ) ;
#14765=CARTESIAN_POINT ( 'NONE',  ( 39.99999999999998579, 8.000000000000000000, -29.99999999999999645 ) ) ;
#14769=ORIENTED_EDGE ( 'NONE', *, *, #16461, .T. ) ;
#14789=EDGE_CURVE ( 'NONE', #9130, #2208, #12614, .T. ) ;
#14819=VERTEX_POINT ( 'NONE', #753 ) ;
#14827=ORIENTED_EDGE ( 'NONE', *, *, #10226, .F. ) ;
#14843=CARTESIAN_POINT ( 'NONE',  ( -40.00000000000000000, 8.000000000000000000, -30.00000000000000355 ) ) ;
#14846=CARTESIAN_POINT ( 'NONE',  ( 39.99999999999998579, 0.000000000000000000, 39.99999999999998579 ) ) ;
#14872=PLANE ( 'NONE',  #850 ) ;
#14878=CIRCLE ( 'NONE', #14320, 4.999999999999997335 ) ;
#14882=DIRECTION ( 'NONE',  ( 0.000000000000000000, -1.000000000000000000, 0.000000000000000000 ) ) ;
#14946=PLANE ( 'NONE',  #3274 ) ;
#14956=AXIS2_PLACEMENT_3D ( 'NONE', #12980, #15548, #8645 ) ;
#14976=CARTESIAN_POINT ( 'NONE',  ( 39.99999999999998579, -20.00000000000000000, 39.99999999999998579 ) ) ;
#15017=VECTOR ( 'NONE', #2603, 1000.000000000000000 ) ;
#15019=CARTESIAN_POINT ( 'NONE',  ( -40.00000000000000000, 4.000000000000000000, -30.00000000000000000 ) ) ;
#15021=CARTESIAN_POINT ( 'NONE',  ( 39.99999999999998579, 0.000000000000000000, 33.00000000000001421 ) ) ;
#15042=VERTEX_POINT ( 'NONE', #11354 ) ;
#15094=EDGE_CURVE ( 'NONE', #4421, #2973, #13753, .T. ) ;
#15158=ADVANCED_FACE ( 'NONE', ( #7189 ), #4365, .T. ) ;
#15163=VECTOR ( 'NONE', #13996, 1000.000000000000000 ) ;
#15232=CARTESIAN_POINT ( 'NONE',  ( 39.99999999999998579, 4.000000000000000000, -30.00000000000000000 ) ) ;
#15298=EDGE_CURVE ( 'NONE', #2717, #11143, #14406, .T. ) ;
#15301=ORIENTED_EDGE ( 'NONE', *, *, #5126, .T. ) ;
#15344=DIRECTION ( 'NONE',  ( 8.673617379884036705E-17, -8.673617379884037444E-16, -1.000000000000000000 ) ) ;
#15357=ORIENTED_EDGE ( 'NONE', *, *, #612, .F. ) ;
#15384=CARTESIAN_POINT ( 'NONE',  ( 39.99999999999998579, 5.659323622547703371E-16, -33.00000000000000000 ) ) ;
#15465=DIRECTION ( 'NONE',  ( 0.000000000000000000, 1.000000000000000000, 0.000000000000000000 ) ) ;
#15479=LINE ( 'NONE', #15384, #6465 ) ;
#15495=EDGE_CURVE ( 'NONE', #10480, #11460, #7767, .T. ) ;
#15498=PRODUCT ( 'Detachable Battery Pack Module', 'Detachable Battery Pack Module', '', ( #5621 ) ) ;
#15548=DIRECTION ( 'NONE',  ( 1.000000000000000000, -0.000000000000000000, 0.000000000000000000 ) ) ;
#15569=CARTESIAN_POINT ( 'NONE',  ( 39.99999999999999289, 8.000000000000000000, -39.99999999999999289 ) ) ;
#15662=LINE ( 'NONE', #7607, #9022 ) ;
#15674=ORIENTED_EDGE ( 'NONE', *, *, #14584, .F. ) ;
#15739=VERTEX_POINT ( 'NONE', #16796 ) ;
#15748=CARTESIAN_POINT ( 'NONE',  ( 39.99999999999998579, -20.00000000000000000, 39.99999999999998579 ) ) ;
#15785=ORIENTED_EDGE ( 'NONE', *, *, #11729, .T. ) ;
#15850=ADVANCED_FACE ( 'NONE', ( #9155 ), #6513, .F. ) ;
#15878=ORIENTED_EDGE ( 'NONE', *, *, #8063, .F. ) ;
#15888=UNCERTAINTY_MEASURE_WITH_UNIT (LENGTH_MEASURE( 1.000000000000000082E-05 ), #8472, 'distance_accuracy_value', 'NONE');
#15971=PLANE ( 'NONE',  #3899 ) ;
#15998=DIRECTION ( 'NONE',  ( 0.000000000000000000, 1.000000000000000000, 0.000000000000000000 ) ) ;
#16020=VERTEX_POINT ( 'NONE', #5871 ) ;
#16029=DIRECTION ( 'NONE',  ( -1.541976423090495387E-16, 0.000000000000000000, -1.000000000000000000 ) ) ;
#16049=CARTESIAN_POINT ( 'NONE',  ( 39.99999999999998579, 4.000000000000000000, -33.00000000000000000 ) ) ;
#16068=VECTOR ( 'NONE', #1893, 1000.000000000000000 ) ;
#16103=EDGE_CURVE ( 'NONE', #925, #14757, #16590, .T. ) ;
#16111=AXIS2_PLACEMENT_3D ( 'NONE', #14194, #9122, #14525 ) ;
#16140=DIRECTION ( 'NONE',  ( -0.000000000000000000, -1.000000000000000000, -0.000000000000000000 ) ) ;
#16152=CARTESIAN_POINT ( 'NONE',  ( 34.99999999999999289, 8.000000000000000000, -39.99999999999999289 ) ) ;
#16182=EDGE_CURVE ( 'NONE', #14819, #11143, #7451, .T. ) ;
#16213=DIRECTION ( 'NONE',  ( 8.673617379884036705E-17, -0.000000000000000000, -1.000000000000000000 ) ) ;
#16253=ADVANCED_FACE ( 'NONE', ( #982 ), #2671, .T. ) ;
#16260=DIRECTION ( 'NONE',  ( -8.673617379884036705E-17, 0.000000000000000000, 1.000000000000000000 ) ) ;
#16346=PRODUCT_DEFINITION_SHAPE ( 'NONE', 'NONE',  #17347 ) ;
#16357=ADVANCED_FACE ( 'NONE', ( #5682 ), #11069, .T. ) ;
#16374=VECTOR ( 'NONE', #2541, 1000.000000000000000 ) ;
#16377=ORIENTED_EDGE ( 'NONE', *, *, #14565, .F. ) ;
#16388=FACE_OUTER_BOUND ( 'NONE', #12357, .T. ) ;
#16398=EDGE_LOOP ( 'NONE', ( #9478, #8153, #6685, #8952 ) ) ;
#16403=EDGE_LOOP ( 'NONE', ( #14769, #1453, #480, #4021 ) ) ;
#16405=AXIS2_PLACEMENT_3D ( 'NONE', #3777, #17237, #11919 ) ;
#16417=VECTOR ( 'NONE', #5313, 1000.000000000000000 ) ;
#16456=DIRECTION ( 'NONE',  ( 7.523163845262643335E-32, -1.000000000000000000, -8.673617379884037444E-16 ) ) ;
#16458=LINE ( 'NONE', #14846, #17468 ) ;
#16461=EDGE_CURVE ( 'NONE', #4201, #6776, #11414, .T. ) ;
#16468=SURFACE_SIDE_STYLE ('',( #5662 ) ) ;
#16475=DIRECTION ( 'NONE',  ( 0.000000000000000000, -0.000000000000000000, 1.000000000000000000 ) ) ;
#16485=DIRECTION ( 'NONE',  ( 0.000000000000000000, 0.000000000000000000, -1.000000000000000000 ) ) ;
#16555=CIRCLE ( 'NONE', #12295, 4.999999999999997335 ) ;
#16560=AXIS2_PLACEMENT_3D ( 'NONE', #13147, #6420, #10305 ) ;
#16585=ORIENTED_EDGE ( 'NONE', *, *, #3557, .F. ) ;
#16590=LINE ( 'NONE', #2142, #6947 ) ;
#16598=MECHANICAL_DESIGN_GEOMETRIC_PRESENTATION_REPRESENTATION('',(#1372),#3913);
#16626=LINE ( 'NONE', #14843, #8999 ) ;
#16679=ORIENTED_EDGE ( 'NONE', *, *, #302, .T. ) ;
#16729=CARTESIAN_POINT ( 'NONE',  ( 39.99999999999998579, -20.00000000000000000, -35.00000000000002132 ) ) ;
#16742=EDGE_CURVE ( 'NONE', #1481, #1803, #2096, .T. ) ;
#16765=CARTESIAN_POINT ( 'NONE',  ( 39.99999999999998579, 4.000000000000000000, -30.00000000000000000 ) ) ;
#16796=CARTESIAN_POINT ( 'NONE',  ( 39.99999999999998579, 8.000000000000007105, 30.00000000000001066 ) ) ;
#16909=EDGE_CURVE ( 'NONE', #11936, #14757, #12008, .T. ) ;
#16917=EDGE_LOOP ( 'NONE', ( #9015, #14827, #12921, #9261 ) ) ;
#16964=VECTOR ( 'NONE', #12009, 1000.000000000000000 ) ;
#16988=AXIS2_PLACEMENT_3D ( 'NONE', #3137, #15344, #7122 ) ;
#17035=CARTESIAN_POINT ( 'NONE',  ( 39.99999999999998579, 8.000000000000007105, 30.00000000000001066 ) ) ;
#17052=CARTESIAN_POINT ( 'NONE',  ( 39.99999999999998579, 4.000000000000000000, -30.00000000000000000 ) ) ;
#17073=SHAPE_REPRESENTATION ( 'Detachable Battery Pack Module', ( #3583 ), #803 ) ;
#17110=COLOUR_RGB ( '', 0.09019608, 0.27058824, 0.51372549) ;
#17134=LINE ( 'NONE', #11650, #16374 ) ;
#17233=ADVANCED_FACE ( 'NONE', ( #6504 ), #15971, .T. ) ;
#17237=DIRECTION ( 'NONE',  ( 0.000000000000000000, 1.000000000000000000, 0.000000000000000000 ) ) ;
#17250=LINE ( 'NONE', #7858, #1694 ) ;
#17323=DIRECTION ( 'NONE',  ( -1.000000000000000000, 0.000000000000000000, -8.673617379884037937E-17 ) ) ;
#17338=ORIENTED_EDGE ( 'NONE', *, *, #14789, .T. ) ;
#17347=PRODUCT_DEFINITION ( 'UNKNOWN', '', #3897, #6956 ) ;
#17364=VERTEX_POINT ( 'NONE', #10111 ) ;
#17381=AXIS2_PLACEMENT_3D ( 'NONE', #12239, #109, #10822 ) ;
#17407=DIRECTION ( 'NONE',  ( 6.938893903907229364E-16, -0.000000000000000000, -1.000000000000000000 ) ) ;
#17440=LINE ( 'NONE', #7775, #16417 ) ;
#17441=VECTOR ( 'NONE', #3258, 1000.000000000000000 ) ;
#17468=VECTOR ( 'NONE', #4321, 1000.000000000000000 ) ;
#17472=CARTESIAN_POINT ( 'NONE',  ( 39.99999999999998579, -20.00000000000000000, 34.99999999999999289 ) ) ;
ENDSEC;
END-ISO-10303-21;
